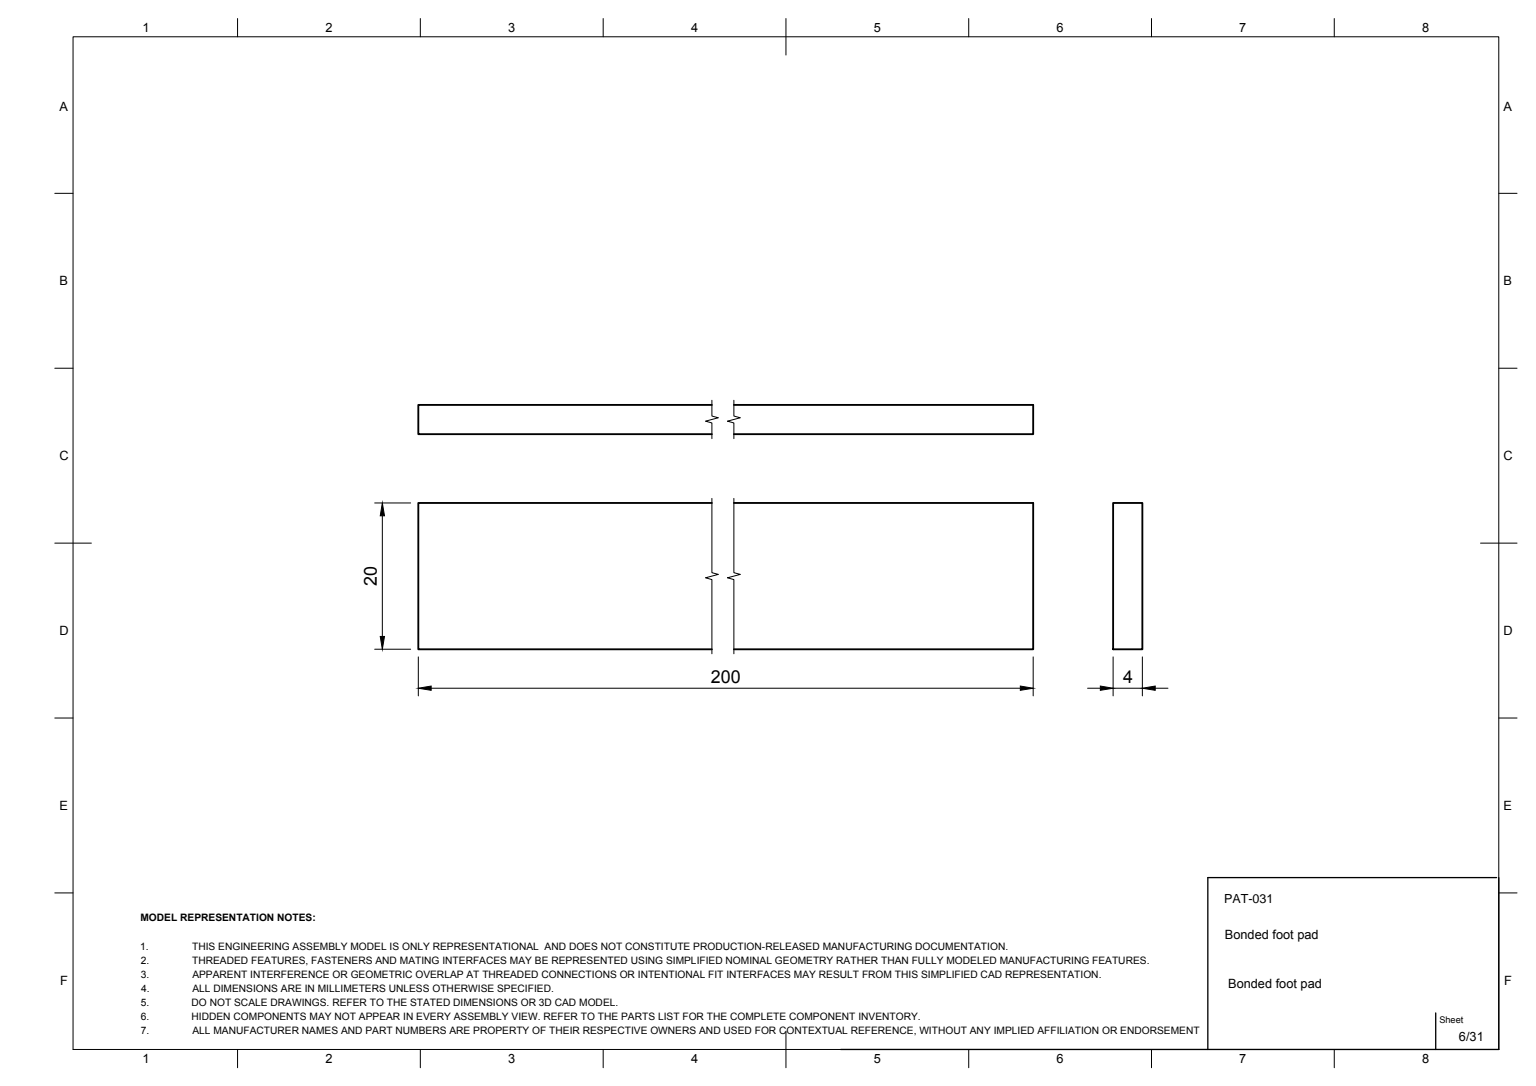
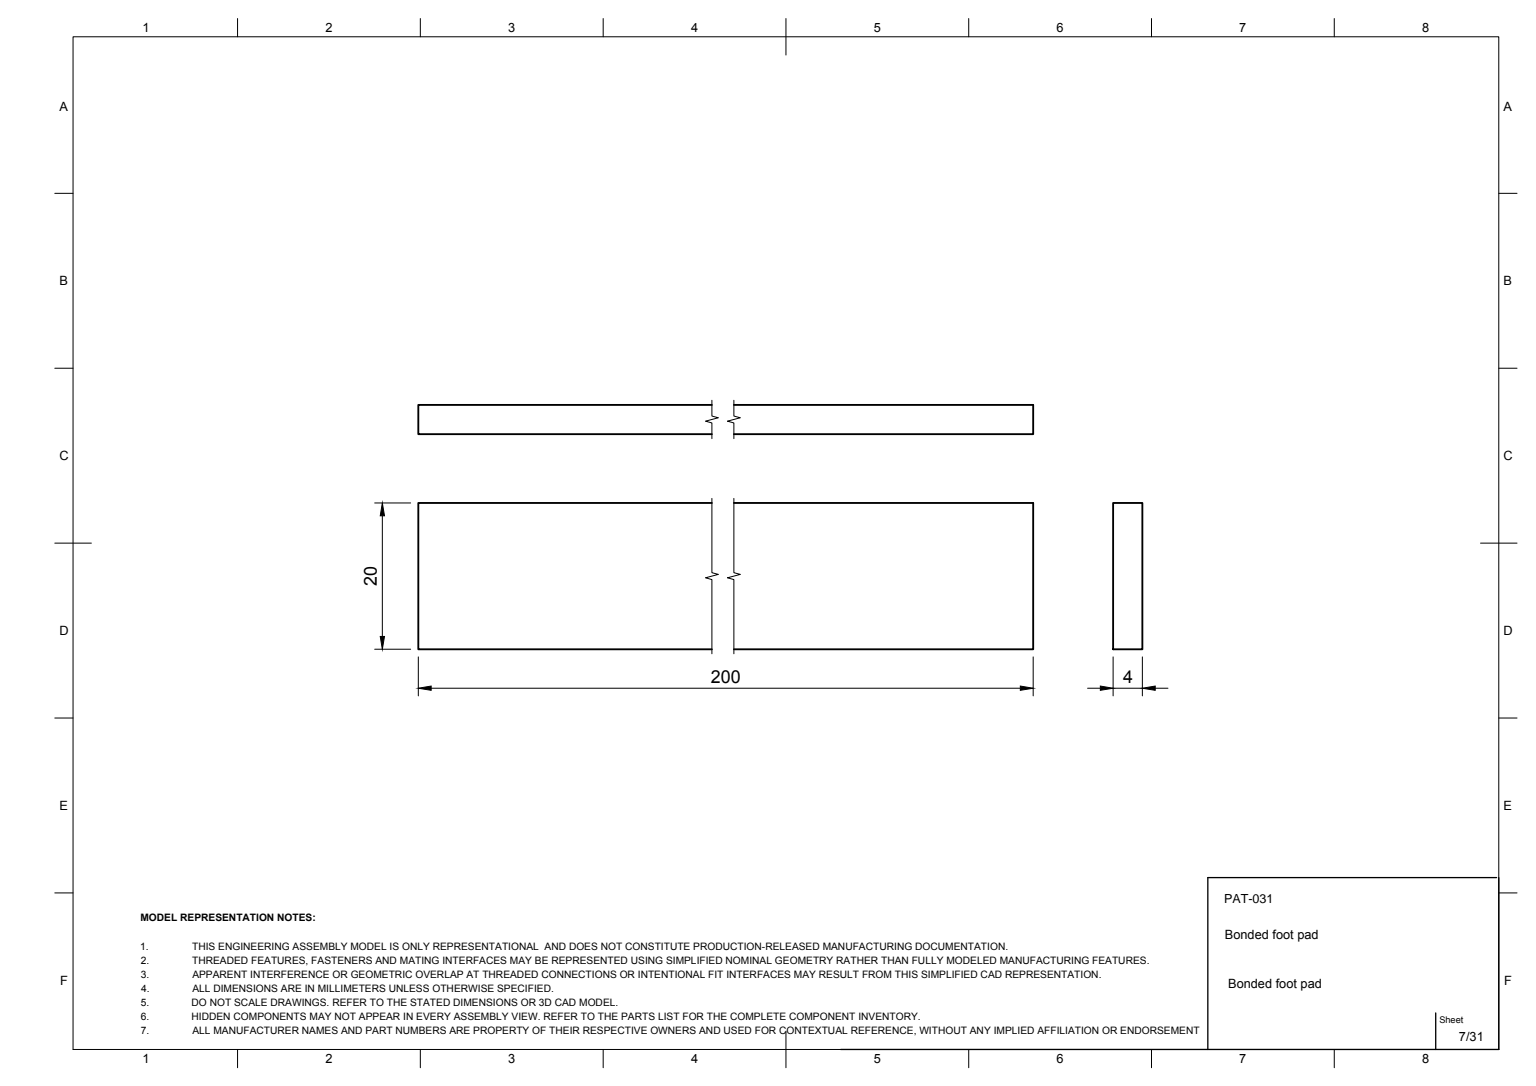
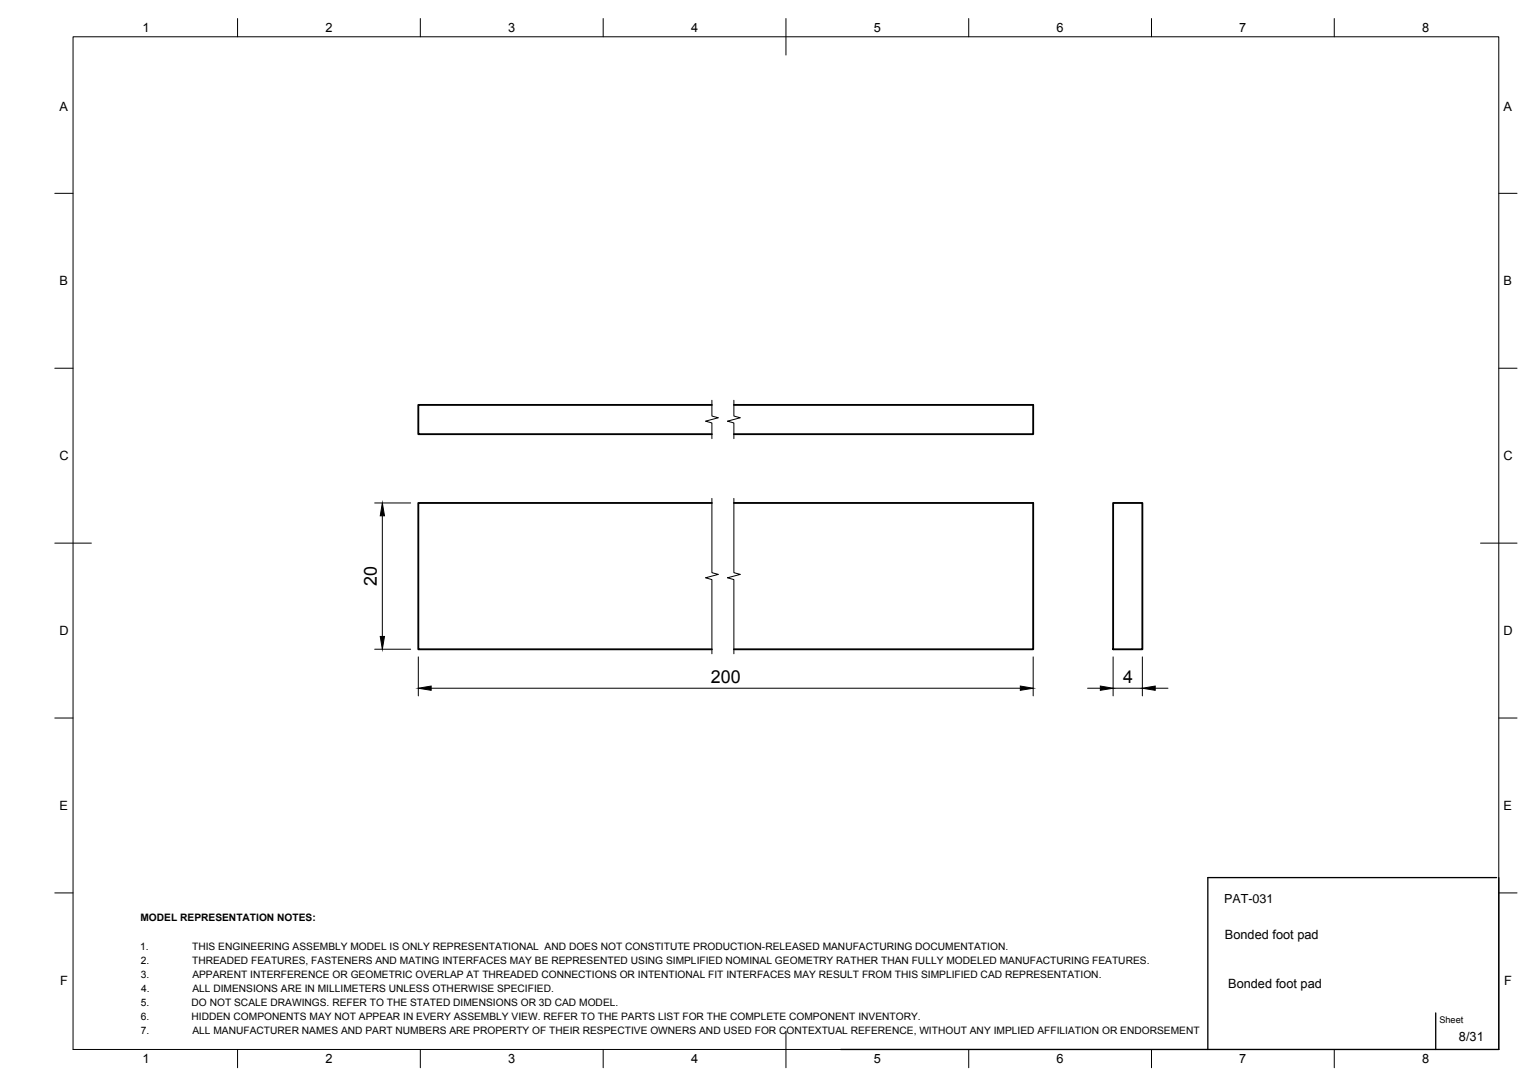
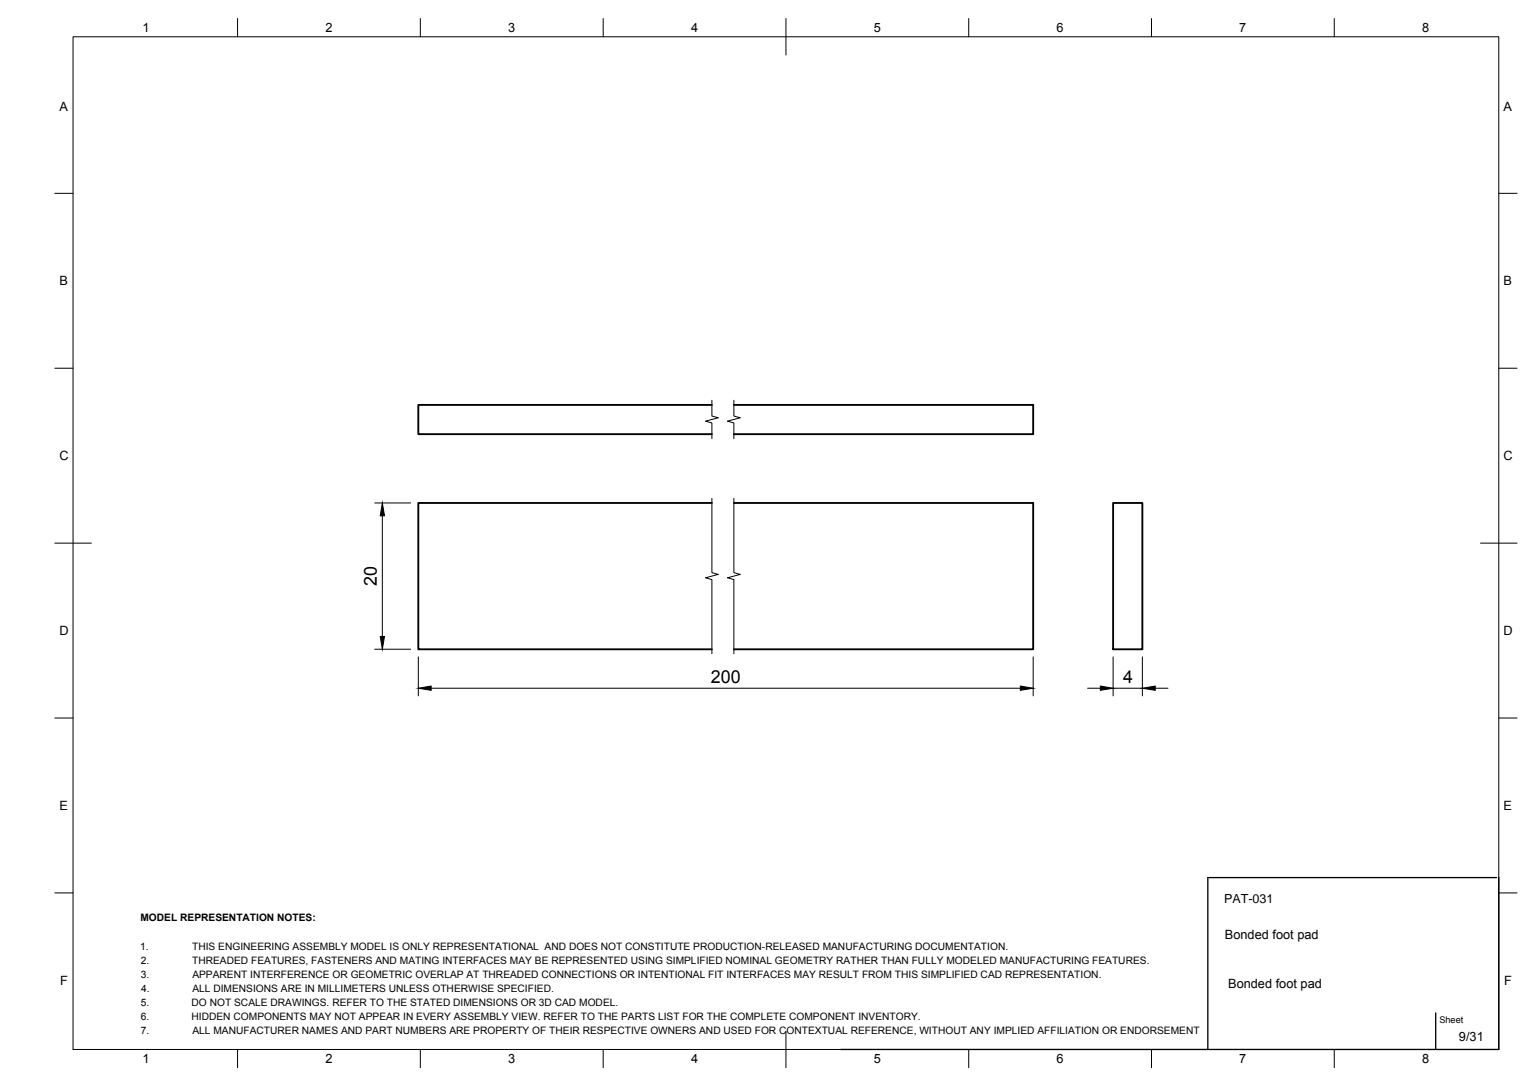
ISO-10303-21;
HEADER;
/* Generated by software containing ST-Developer
 * from STEP Tools, Inc. (www.steptools.com) 
 */

FILE_DESCRIPTION(
/* description */ ('Double-row support with tensioned shaft'),
/* implementation_level */ '2;1');

FILE_NAME(
/* name */ 'Bonded foot pad.step',
/* time_stamp */ '2026-10-27T10:50:35-07:00',
/* author */ (''),
/* organization */ (''),
/* preprocessor_version */ 'ST-DEVELOPER v20.2',
/* originating_system */ 'Autodesk Translation Framework v15.17.0.0',
/* authorisation */ '');

FILE_SCHEMA (('AUTOMOTIVE_DESIGN { 1 0 10303 214 3 1 1 }'));
ENDSEC;

DATA;
#10=MECHANICAL_DESIGN_GEOMETRIC_PRESENTATION_REPRESENTATION('',(#480),#11559);
#416=SHAPE_REPRESENTATION_RELATIONSHIP('SRR','None',#11724,#448);
#448=ADVANCED_BREP_SHAPE_REPRESENTATION('',(#513),#11526);
#480=STYLED_ITEM('',(#11960),#513);
#513=MANIFOLD_SOLID_BREP('Body1',#6325);
#685=PLANE('',#6759);
#686=PLANE('',#6760);
#687=PLANE('',#6761);
#688=PLANE('',#6762);
#689=PLANE('',#6763);
#690=PLANE('',#6764);
#935=FACE_OUTER_BOUND('',#1303,.T.);
#936=FACE_OUTER_BOUND('',#1304,.T.);
#937=FACE_OUTER_BOUND('',#1305,.T.);
#938=FACE_OUTER_BOUND('',#1306,.T.);
#939=FACE_OUTER_BOUND('',#1307,.T.);
#940=FACE_OUTER_BOUND('',#1308,.T.);
#1303=EDGE_LOOP('',(#4426,#4427,#4428,#4429));
#1304=EDGE_LOOP('',(#4430,#4431,#4432,#4433));
#1305=EDGE_LOOP('',(#4434,#4435,#4436,#4437));
#1306=EDGE_LOOP('',(#4438,#4439,#4440,#4441));
#1307=EDGE_LOOP('',(#4442,#4443,#4444,#4445));
#1308=EDGE_LOOP('',(#4446,#4447,#4448,#4449));
#1766=LINE('',#9339,#2313);
#1767=LINE('',#9341,#2314);
#1768=LINE('',#9343,#2315);
#1769=LINE('',#9344,#2316);
#1770=LINE('',#9347,#2317);
#1771=LINE('',#9349,#2318);
#1772=LINE('',#9350,#2319);
#1773=LINE('',#9353,#2320);
#1774=LINE('',#9355,#2321);
#1775=LINE('',#9356,#2322);
#1776=LINE('',#9358,#2323);
#1777=LINE('',#9359,#2324);
#2313=VECTOR('',#7489,1.);
#2314=VECTOR('',#7490,1.);
#2315=VECTOR('',#7491,1.);
#2316=VECTOR('',#7492,1.);
#2317=VECTOR('',#7495,1.);
#2318=VECTOR('',#7496,1.);
#2319=VECTOR('',#7497,1.);
#2320=VECTOR('',#7500,1.);
#2321=VECTOR('',#7501,1.);
#2322=VECTOR('',#7502,1.);
#2323=VECTOR('',#7505,1.);
#2324=VECTOR('',#7506,1.);
#3059=VERTEX_POINT('',#9337);
#3060=VERTEX_POINT('',#9338);
#3061=VERTEX_POINT('',#9340);
#3062=VERTEX_POINT('',#9342);
#3063=VERTEX_POINT('',#9346);
#3064=VERTEX_POINT('',#9348);
#3065=VERTEX_POINT('',#9352);
#3066=VERTEX_POINT('',#9354);
#3598=EDGE_CURVE('',#3059,#3060,#1766,.T.);
#3599=EDGE_CURVE('',#3060,#3061,#1767,.T.);
#3600=EDGE_CURVE('',#3062,#3061,#1768,.T.);
#3601=EDGE_CURVE('',#3059,#3062,#1769,.T.);
#3602=EDGE_CURVE('',#3063,#3059,#1770,.T.);
#3603=EDGE_CURVE('',#3064,#3062,#1771,.T.);
#3604=EDGE_CURVE('',#3063,#3064,#1772,.T.);
#3605=EDGE_CURVE('',#3065,#3063,#1773,.T.);
#3606=EDGE_CURVE('',#3066,#3064,#1774,.T.);
#3607=EDGE_CURVE('',#3065,#3066,#1775,.T.);
#3608=EDGE_CURVE('',#3060,#3065,#1776,.T.);
#3609=EDGE_CURVE('',#3061,#3066,#1777,.T.);
#4426=ORIENTED_EDGE('',*,*,#3598,.T.);
#4427=ORIENTED_EDGE('',*,*,#3599,.T.);
#4428=ORIENTED_EDGE('',*,*,#3600,.F.);
#4429=ORIENTED_EDGE('',*,*,#3601,.F.);
#4430=ORIENTED_EDGE('',*,*,#3602,.T.);
#4431=ORIENTED_EDGE('',*,*,#3601,.T.);
#4432=ORIENTED_EDGE('',*,*,#3603,.F.);
#4433=ORIENTED_EDGE('',*,*,#3604,.F.);
#4434=ORIENTED_EDGE('',*,*,#3605,.T.);
#4435=ORIENTED_EDGE('',*,*,#3604,.T.);
#4436=ORIENTED_EDGE('',*,*,#3606,.F.);
#4437=ORIENTED_EDGE('',*,*,#3607,.F.);
#4438=ORIENTED_EDGE('',*,*,#3608,.T.);
#4439=ORIENTED_EDGE('',*,*,#3607,.T.);
#4440=ORIENTED_EDGE('',*,*,#3609,.F.);
#4441=ORIENTED_EDGE('',*,*,#3599,.F.);
#4442=ORIENTED_EDGE('',*,*,#3609,.T.);
#4443=ORIENTED_EDGE('',*,*,#3606,.T.);
#4444=ORIENTED_EDGE('',*,*,#3603,.T.);
#4445=ORIENTED_EDGE('',*,*,#3600,.T.);
#4446=ORIENTED_EDGE('',*,*,#3608,.F.);
#4447=ORIENTED_EDGE('',*,*,#3598,.F.);
#4448=ORIENTED_EDGE('',*,*,#3602,.F.);
#4449=ORIENTED_EDGE('',*,*,#3605,.F.);
#5998=ADVANCED_FACE('',(#935),#685,.T.);
#5999=ADVANCED_FACE('',(#936),#686,.T.);
#6000=ADVANCED_FACE('',(#937),#687,.T.);
#6001=ADVANCED_FACE('',(#938),#688,.T.);
#6002=ADVANCED_FACE('',(#939),#689,.T.);
#6003=ADVANCED_FACE('',(#940),#690,.F.);
#6325=CLOSED_SHELL('',(#5998,#5999,#6000,#6001,#6002,#6003));
#6758=AXIS2_PLACEMENT_3D('',#9335,#7485,#7486);
#6759=AXIS2_PLACEMENT_3D('',#9336,#7487,#7488);
#6760=AXIS2_PLACEMENT_3D('',#9345,#7493,#7494);
#6761=AXIS2_PLACEMENT_3D('',#9351,#7498,#7499);
#6762=AXIS2_PLACEMENT_3D('',#9357,#7503,#7504);
#6763=AXIS2_PLACEMENT_3D('',#9360,#7507,#7508);
#6764=AXIS2_PLACEMENT_3D('',#9361,#7509,#7510);
#7485=DIRECTION('axis',(0.,0.,1.));
#7486=DIRECTION('refdir',(1.,0.,0.));
#7487=DIRECTION('center_axis',(0.,1.,0.));
#7488=DIRECTION('ref_axis',(-1.,0.,0.));
#7489=DIRECTION('',(-1.,0.,0.));
#7490=DIRECTION('',(0.,0.,1.));
#7491=DIRECTION('',(-1.,0.,0.));
#7492=DIRECTION('',(0.,0.,1.));
#7493=DIRECTION('center_axis',(1.,0.,0.));
#7494=DIRECTION('ref_axis',(0.,1.,0.));
#7495=DIRECTION('',(0.,1.,0.));
#7496=DIRECTION('',(0.,1.,0.));
#7497=DIRECTION('',(0.,0.,1.));
#7498=DIRECTION('center_axis',(0.,-1.,0.));
#7499=DIRECTION('ref_axis',(1.,0.,0.));
#7500=DIRECTION('',(1.,0.,0.));
#7501=DIRECTION('',(1.,0.,0.));
#7502=DIRECTION('',(0.,0.,1.));
#7503=DIRECTION('center_axis',(-1.,0.,0.));
#7504=DIRECTION('ref_axis',(0.,-1.,0.));
#7505=DIRECTION('',(0.,-1.,0.));
#7506=DIRECTION('',(0.,-1.,0.));
#7507=DIRECTION('center_axis',(0.,0.,1.));
#7508=DIRECTION('ref_axis',(1.,0.,0.));
#7509=DIRECTION('center_axis',(0.,0.,1.));
#7510=DIRECTION('ref_axis',(1.,0.,0.));
#9335=CARTESIAN_POINT('',(0.,0.,0.));
#9336=CARTESIAN_POINT('Origin',(10.,-2.,-0.4));
#9337=CARTESIAN_POINT('',(10.,-2.,-0.4));
#9338=CARTESIAN_POINT('',(-10.,-2.,-0.4));
#9339=CARTESIAN_POINT('',(10.,-2.,-0.4));
#9340=CARTESIAN_POINT('',(-10.,-2.,0.));
#9341=CARTESIAN_POINT('',(-10.,-2.,-0.4));
#9342=CARTESIAN_POINT('',(10.,-2.,0.));
#9343=CARTESIAN_POINT('',(10.,-2.,0.));
#9344=CARTESIAN_POINT('',(10.,-2.,-0.4));
#9345=CARTESIAN_POINT('Origin',(10.,-4.,-0.4));
#9346=CARTESIAN_POINT('',(10.,-4.,-0.4));
#9347=CARTESIAN_POINT('',(10.,-4.,-0.4));
#9348=CARTESIAN_POINT('',(10.,-4.,0.));
#9349=CARTESIAN_POINT('',(10.,-4.,0.));
#9350=CARTESIAN_POINT('',(10.,-4.,-0.4));
#9351=CARTESIAN_POINT('Origin',(-10.,-4.,-0.4));
#9352=CARTESIAN_POINT('',(-10.,-4.,-0.4));
#9353=CARTESIAN_POINT('',(-10.,-4.,-0.4));
#9354=CARTESIAN_POINT('',(-10.,-4.,0.));
#9355=CARTESIAN_POINT('',(-10.,-4.,0.));
#9356=CARTESIAN_POINT('',(-10.,-4.,-0.4));
#9357=CARTESIAN_POINT('Origin',(-10.,-2.,-0.4));
#9358=CARTESIAN_POINT('',(-10.,-2.,-0.4));
#9359=CARTESIAN_POINT('',(-10.,-2.,0.));
#9360=CARTESIAN_POINT('Origin',(0.,-3.,0.));
#9361=CARTESIAN_POINT('Origin',(0.,-3.,-0.4));
#11489=UNCERTAINTY_MEASURE_WITH_UNIT(LENGTH_MEASURE(0.001),#11560,
'DISTANCE_ACCURACY_VALUE',
'Maximum model space distance between geometric entities at asserted c
onnectivities');
#11522=UNCERTAINTY_MEASURE_WITH_UNIT(LENGTH_MEASURE(0.001),#11560,
'DISTANCE_ACCURACY_VALUE',
'Maximum model space distance between geometric entities at asserted c
onnectivities');
#11526=(
GEOMETRIC_REPRESENTATION_CONTEXT(3)
GLOBAL_UNCERTAINTY_ASSIGNED_CONTEXT((#11489))
GLOBAL_UNIT_ASSIGNED_CONTEXT((#11560,#11562,#11563))
REPRESENTATION_CONTEXT('','3D')
);
#11559=(
GEOMETRIC_REPRESENTATION_CONTEXT(3)
GLOBAL_UNCERTAINTY_ASSIGNED_CONTEXT((#11522))
GLOBAL_UNIT_ASSIGNED_CONTEXT((#11560,#11562,#11563))
REPRESENTATION_CONTEXT('','3D')
);
#11560=(
LENGTH_UNIT()
NAMED_UNIT(*)
SI_UNIT(.CENTI.,.METRE.)
);
#11562=(
NAMED_UNIT(*)
PLANE_ANGLE_UNIT()
SI_UNIT($,.RADIAN.)
);
#11563=(
NAMED_UNIT(*)
SI_UNIT($,.STERADIAN.)
SOLID_ANGLE_UNIT()
);
#11567=SHAPE_DEFINITION_REPRESENTATION(#11603,#11724);
#11603=PRODUCT_DEFINITION_SHAPE('',$,#11761);
#11724=SHAPE_REPRESENTATION('',(#6758),#11526);
#11757=PRODUCT_DEFINITION_CONTEXT('part definition',#11867,'design');
#11761=PRODUCT_DEFINITION('Bonded foot pad','Bonded foot pad',#11797,#11757);
#11797=PRODUCT_DEFINITION_FORMATION('',$,#11872);
#11867=APPLICATION_CONTEXT(
'Core Data for Automotive Mechanical Design Process');
#11868=PRODUCT_CONTEXT('part definition',#11867,'mechanical');
#11872=PRODUCT('Bonded foot pad','Bonded foot pad','Bonded foot pad',(#11868));
#11954=COLOUR_RGB('Sky Blue',0.24,0.69,0.87);
#11955=FILL_AREA_STYLE_COLOUR('',#11954);
#11956=FILL_AREA_STYLE('',(#11955));
#11957=SURFACE_STYLE_FILL_AREA(#11956);
#11958=SURFACE_SIDE_STYLE('',(#11957));
#11959=SURFACE_STYLE_USAGE(.BOTH.,#11958);
#11960=PRESENTATION_STYLE_ASSIGNMENT((#11959));
ENDSEC;
END-ISO-10303-21;
